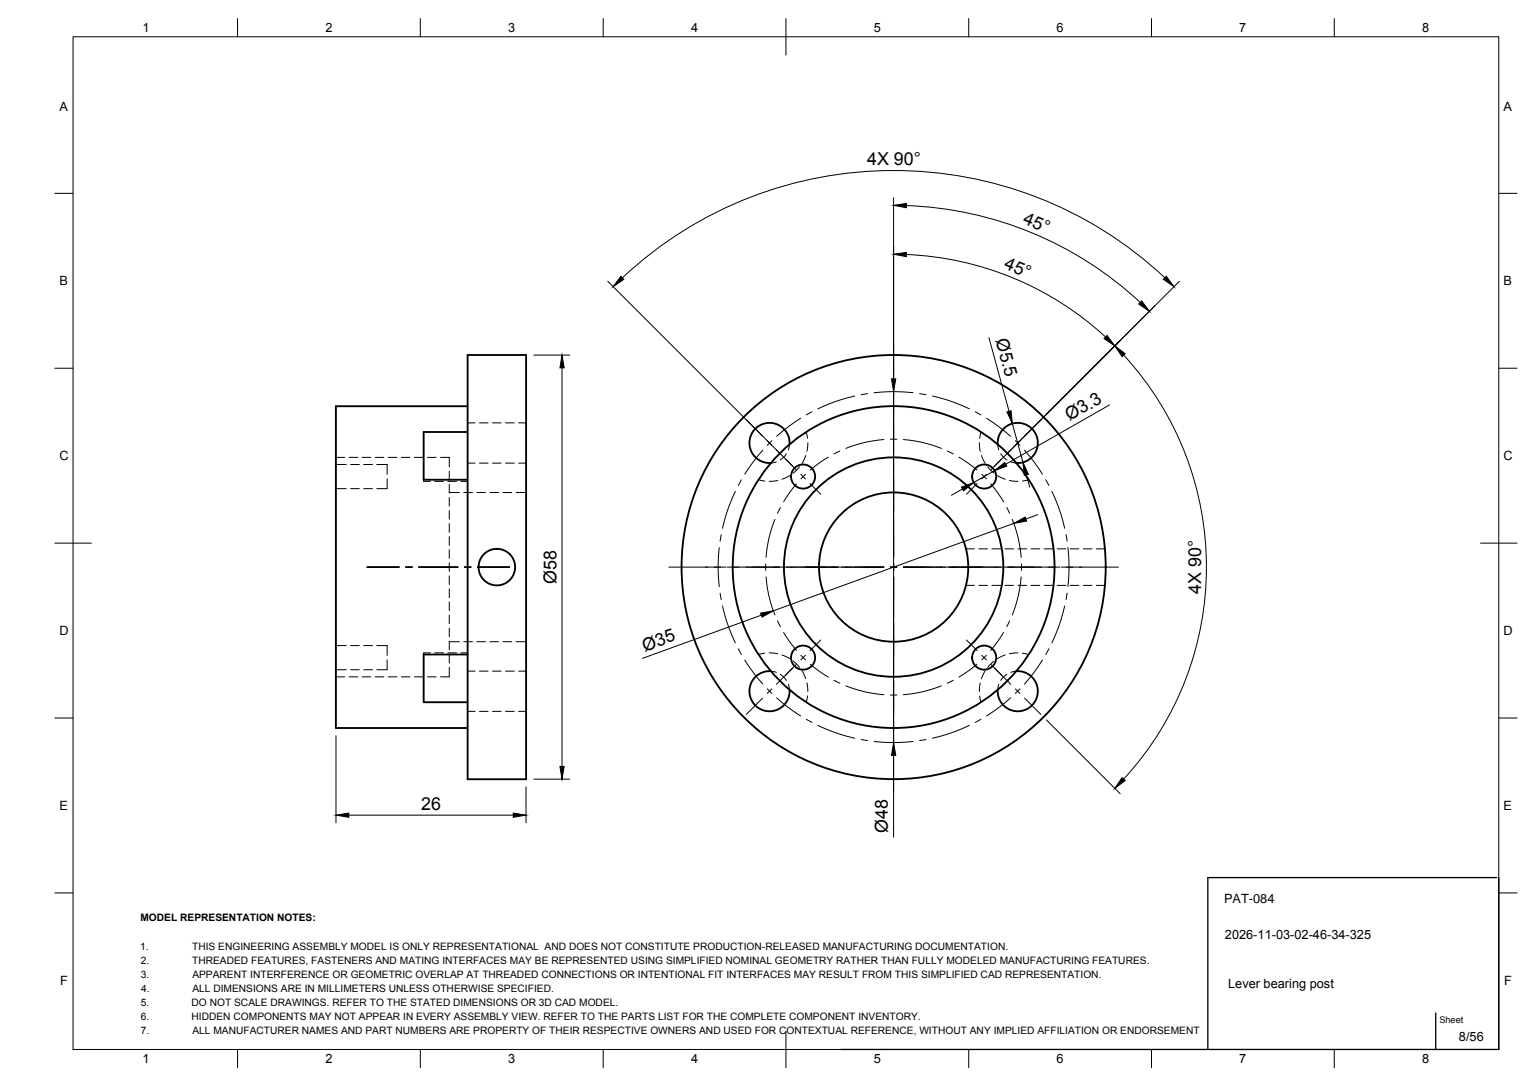
ISO-10303-21;
HEADER;
/* Generated by software containing ST-Developer
 * from STEP Tools, Inc. (www.steptools.com) 
 */

FILE_DESCRIPTION(
/* description */ ('Quick-return (Whitworth) mechanism'),
/* implementation_level */ '2;1');

FILE_NAME(
/* name */ 'Lever bearing post.step',
/* time_stamp */ '2026-10-28T03:25:57-07:00',
/* author */ (''),
/* organization */ (''),
/* preprocessor_version */ 'ST-DEVELOPER v20.2',
/* originating_system */ 'Autodesk Translation Framework v15.17.0.0',
/* authorisation */ '');

FILE_SCHEMA (('AUTOMOTIVE_DESIGN { 1 0 10303 214 3 1 1 }'));
ENDSEC;

DATA;
#10=MECHANICAL_DESIGN_GEOMETRIC_PRESENTATION_REPRESENTATION('',(#493),#14878);
#366=B_SPLINE_CURVE_WITH_KNOTS('',3,(#12105,#12106,#12107,#12108,#12109,
#12110,#12111,#12112,#12113,#12114),.UNSPECIFIED.,.F.,.F.,(4,2,2,2,4),(0.,
0.0945941824764479,0.189188364952896,0.283770357603024,0.378352350253152),
 .UNSPECIFIED.);
#367=B_SPLINE_CURVE_WITH_KNOTS('',3,(#12115,#12116,#12117,#12118,#12119,
#12120,#12121,#12122,#12123,#12124,#12125,#12126,#12127,#12128,#12129,#12130,
#12131,#12132,#12133,#12134,#12135,#12136,#12137,#12138,#12139,#12140),
 .UNSPECIFIED.,.F.,.F.,(4,2,2,2,2,2,2,2,2,2,2,2,4),(0.378352350253152,0.47293434290328,
0.567516335553408,0.662110518029855,0.756704700506303,0.851298882982751,
0.945893065459199,1.04047505810933,1.13505705075946,1.22963904340958,1.32422103605971,
1.41881521853616,1.51340940101261),.UNSPECIFIED.);
#368=B_SPLINE_CURVE_WITH_KNOTS('',3,(#12144,#12145,#12146,#12147,#12148,
#12149,#12150,#12151,#12152,#12153,#12154,#12155,#12156,#12157,#12158,#12159,
#12160,#12161,#12162,#12163,#12164,#12165,#12166,#12167,#12168,#12169),
 .UNSPECIFIED.,.F.,.F.,(4,2,2,2,2,2,2,2,2,2,2,2,4),(0.,0.0942219535700049,
0.18844390714001,0.282665684012033,0.376887460884057,0.471109237756081,
0.565331014628104,0.659552968198109,0.753774921768114,0.847996875338119,
0.942218828908124,1.03644060578015,1.13066238265217),.UNSPECIFIED.);
#369=B_SPLINE_CURVE_WITH_KNOTS('',3,(#12170,#12171,#12172,#12173,#12174,
#12175,#12176,#12177,#12178,#12179),.UNSPECIFIED.,.F.,.F.,(4,2,2,2,4),(1.13066238265217,
1.22488415952419,1.31910593639622,1.41332788996622,1.50754984353623),
 .UNSPECIFIED.);
#405=SHAPE_REPRESENTATION_RELATIONSHIP('SRR','None',#15073,#449);
#449=ADVANCED_BREP_SHAPE_REPRESENTATION('',(#545),#14830);
#493=STYLED_ITEM('',(#15406),#545);
#545=MANIFOLD_SOLID_BREP('Body1',#7847);
#615=FACE_BOUND('',#1585,.T.);
#616=FACE_BOUND('',#1586,.T.);
#617=FACE_BOUND('',#1587,.T.);
#618=FACE_BOUND('',#1588,.T.);
#619=FACE_BOUND('',#1589,.T.);
#620=FACE_BOUND('',#1597,.T.);
#621=FACE_BOUND('',#1599,.T.);
#622=FACE_BOUND('',#1601,.T.);
#623=FACE_BOUND('',#1603,.T.);
#624=FACE_BOUND('',#1604,.T.);
#625=FACE_BOUND('',#1605,.T.);
#626=FACE_BOUND('',#1606,.T.);
#627=FACE_BOUND('',#1607,.T.);
#628=FACE_BOUND('',#1609,.T.);
#629=FACE_BOUND('',#1610,.T.);
#630=FACE_BOUND('',#1611,.T.);
#631=FACE_BOUND('',#1612,.T.);
#632=FACE_BOUND('',#1613,.T.);
#800=PLANE('',#8448);
#801=PLANE('',#8452);
#802=PLANE('',#8456);
#803=PLANE('',#8460);
#804=PLANE('',#8464);
#805=PLANE('',#8469);
#806=PLANE('',#8474);
#807=PLANE('',#8479);
#808=PLANE('',#8481);
#809=PLANE('',#8505);
#810=PLANE('',#8511);
#811=PLANE('',#8512);
#1077=FACE_OUTER_BOUND('',#1567,.T.);
#1078=FACE_OUTER_BOUND('',#1568,.T.);
#1079=FACE_OUTER_BOUND('',#1569,.T.);
#1080=FACE_OUTER_BOUND('',#1570,.T.);
#1081=FACE_OUTER_BOUND('',#1571,.T.);
#1082=FACE_OUTER_BOUND('',#1572,.T.);
#1083=FACE_OUTER_BOUND('',#1573,.T.);
#1084=FACE_OUTER_BOUND('',#1574,.T.);
#1085=FACE_OUTER_BOUND('',#1575,.T.);
#1086=FACE_OUTER_BOUND('',#1576,.T.);
#1087=FACE_OUTER_BOUND('',#1577,.T.);
#1088=FACE_OUTER_BOUND('',#1578,.T.);
#1089=FACE_OUTER_BOUND('',#1579,.T.);
#1090=FACE_OUTER_BOUND('',#1580,.T.);
#1091=FACE_OUTER_BOUND('',#1581,.T.);
#1092=FACE_OUTER_BOUND('',#1582,.T.);
#1093=FACE_OUTER_BOUND('',#1583,.T.);
#1094=FACE_OUTER_BOUND('',#1584,.T.);
#1095=FACE_OUTER_BOUND('',#1590,.T.);
#1096=FACE_OUTER_BOUND('',#1591,.T.);
#1097=FACE_OUTER_BOUND('',#1592,.T.);
#1098=FACE_OUTER_BOUND('',#1593,.T.);
#1099=FACE_OUTER_BOUND('',#1594,.T.);
#1100=FACE_OUTER_BOUND('',#1595,.T.);
#1101=FACE_OUTER_BOUND('',#1596,.T.);
#1102=FACE_OUTER_BOUND('',#1598,.T.);
#1103=FACE_OUTER_BOUND('',#1600,.T.);
#1104=FACE_OUTER_BOUND('',#1602,.T.);
#1105=FACE_OUTER_BOUND('',#1608,.T.);
#1567=EDGE_LOOP('',(#5406,#5407,#5408,#5409,#5410,#5411));
#1568=EDGE_LOOP('',(#5412,#5413,#5414,#5415));
#1569=EDGE_LOOP('',(#5416));
#1570=EDGE_LOOP('',(#5417,#5418,#5419,#5420));
#1571=EDGE_LOOP('',(#5421));
#1572=EDGE_LOOP('',(#5422,#5423,#5424,#5425));
#1573=EDGE_LOOP('',(#5426));
#1574=EDGE_LOOP('',(#5427,#5428,#5429,#5430));
#1575=EDGE_LOOP('',(#5431));
#1576=EDGE_LOOP('',(#5432,#5433,#5434,#5435));
#1577=EDGE_LOOP('',(#5436,#5437));
#1578=EDGE_LOOP('',(#5438,#5439,#5440,#5441));
#1579=EDGE_LOOP('',(#5442,#5443));
#1580=EDGE_LOOP('',(#5444,#5445,#5446,#5447));
#1581=EDGE_LOOP('',(#5448,#5449));
#1582=EDGE_LOOP('',(#5450,#5451,#5452,#5453));
#1583=EDGE_LOOP('',(#5454,#5455));
#1584=EDGE_LOOP('',(#5456));
#1585=EDGE_LOOP('',(#5457,#5458,#5459,#5460,#5461,#5462,#5463,#5464,#5465));
#1586=EDGE_LOOP('',(#5466));
#1587=EDGE_LOOP('',(#5467));
#1588=EDGE_LOOP('',(#5468));
#1589=EDGE_LOOP('',(#5469));
#1590=EDGE_LOOP('',(#5470,#5471,#5472,#5473));
#1591=EDGE_LOOP('',(#5474,#5475,#5476,#5477));
#1592=EDGE_LOOP('',(#5478,#5479,#5480,#5481));
#1593=EDGE_LOOP('',(#5482,#5483,#5484,#5485));
#1594=EDGE_LOOP('',(#5486,#5487,#5488,#5489,#5490,#5491,#5492,#5493,#5494,
#5495,#5496,#5497,#5498,#5499,#5500,#5501,#5502,#5503,#5504,#5505));
#1595=EDGE_LOOP('',(#5506,#5507,#5508,#5509));
#1596=EDGE_LOOP('',(#5510));
#1597=EDGE_LOOP('',(#5511));
#1598=EDGE_LOOP('',(#5512,#5513,#5514,#5515));
#1599=EDGE_LOOP('',(#5516,#5517));
#1600=EDGE_LOOP('',(#5518,#5519,#5520,#5521));
#1601=EDGE_LOOP('',(#5522,#5523));
#1602=EDGE_LOOP('',(#5524));
#1603=EDGE_LOOP('',(#5525));
#1604=EDGE_LOOP('',(#5526));
#1605=EDGE_LOOP('',(#5527));
#1606=EDGE_LOOP('',(#5528));
#1607=EDGE_LOOP('',(#5529));
#1608=EDGE_LOOP('',(#5530));
#1609=EDGE_LOOP('',(#5531));
#1610=EDGE_LOOP('',(#5532));
#1611=EDGE_LOOP('',(#5533));
#1612=EDGE_LOOP('',(#5534));
#1613=EDGE_LOOP('',(#5535));
#2218=LINE('',#12142,#2741);
#2219=LINE('',#12184,#2742);
#2220=LINE('',#12191,#2743);
#2221=LINE('',#12198,#2744);
#2222=LINE('',#12205,#2745);
#2223=LINE('',#12211,#2746);
#2224=LINE('',#12215,#2747);
#2225=LINE('',#12222,#2748);
#2226=LINE('',#12226,#2749);
#2227=LINE('',#12233,#2750);
#2228=LINE('',#12237,#2751);
#2229=LINE('',#12244,#2752);
#2230=LINE('',#12248,#2753);
#2231=LINE('',#12272,#2754);
#2232=LINE('',#12276,#2755);
#2233=LINE('',#12280,#2756);
#2234=LINE('',#12284,#2757);
#2235=LINE('',#12288,#2758);
#2236=LINE('',#12293,#2759);
#2237=LINE('',#12300,#2760);
#2238=LINE('',#12304,#2761);
#2741=VECTOR('',#9567,0.25);
#2742=VECTOR('',#9572,0.165);
#2743=VECTOR('',#9581,0.165);
#2744=VECTOR('',#9590,0.165);
#2745=VECTOR('',#9599,0.165);
#2746=VECTOR('',#9606,1.);
#2747=VECTOR('',#9609,1.);
#2748=VECTOR('',#9618,1.);
#2749=VECTOR('',#9621,1.);
#2750=VECTOR('',#9630,1.);
#2751=VECTOR('',#9633,1.);
#2752=VECTOR('',#9642,1.);
#2753=VECTOR('',#9645,1.);
#2754=VECTOR('',#9678,0.275);
#2755=VECTOR('',#9683,0.275);
#2756=VECTOR('',#9688,0.275);
#2757=VECTOR('',#9693,0.275);
#2758=VECTOR('',#9698,2.2);
#2759=VECTOR('',#9703,1.5);
#2760=VECTOR('',#9712,2.9);
#2761=VECTOR('',#9717,1.02);
#3240=CIRCLE('',#8446,0.165);
#3241=CIRCLE('',#8447,0.165);
#3242=CIRCLE('',#8450,0.165);
#3243=CIRCLE('',#8451,0.165);
#3244=CIRCLE('',#8454,0.165);
#3245=CIRCLE('',#8455,0.165);
#3246=CIRCLE('',#8458,0.165);
#3247=CIRCLE('',#8459,0.165);
#3248=CIRCLE('',#8462,0.525);
#3249=CIRCLE('',#8463,0.525);
#3250=CIRCLE('',#8465,2.2);
#3251=CIRCLE('',#8467,0.525);
#3252=CIRCLE('',#8468,0.525);
#3253=CIRCLE('',#8470,2.2);
#3254=CIRCLE('',#8472,0.525);
#3255=CIRCLE('',#8473,0.525);
#3256=CIRCLE('',#8475,2.2);
#3257=CIRCLE('',#8477,0.525);
#3258=CIRCLE('',#8478,0.525);
#3259=CIRCLE('',#8480,2.2);
#3260=CIRCLE('',#8482,2.9);
#3261=CIRCLE('',#8483,2.2);
#3262=CIRCLE('',#8484,2.2);
#3263=CIRCLE('',#8485,2.2);
#3264=CIRCLE('',#8486,2.2);
#3265=CIRCLE('',#8487,2.2);
#3266=CIRCLE('',#8488,0.275);
#3267=CIRCLE('',#8489,0.275);
#3268=CIRCLE('',#8490,0.275);
#3269=CIRCLE('',#8491,0.275);
#3270=CIRCLE('',#8493,0.275);
#3271=CIRCLE('',#8495,0.275);
#3272=CIRCLE('',#8497,0.275);
#3273=CIRCLE('',#8499,0.275);
#3274=CIRCLE('',#8501,2.2);
#3275=CIRCLE('',#8503,1.5);
#3276=CIRCLE('',#8504,1.5);
#3277=CIRCLE('',#8506,1.02);
#3278=CIRCLE('',#8508,2.9);
#3279=CIRCLE('',#8510,1.02);
#3679=VERTEX_POINT('',#12103);
#3680=VERTEX_POINT('',#12104);
#3681=VERTEX_POINT('',#12141);
#3682=VERTEX_POINT('',#12143);
#3683=VERTEX_POINT('',#12181);
#3684=VERTEX_POINT('',#12183);
#3685=VERTEX_POINT('',#12188);
#3686=VERTEX_POINT('',#12190);
#3687=VERTEX_POINT('',#12195);
#3688=VERTEX_POINT('',#12197);
#3689=VERTEX_POINT('',#12202);
#3690=VERTEX_POINT('',#12204);
#3691=VERTEX_POINT('',#12209);
#3692=VERTEX_POINT('',#12210);
#3693=VERTEX_POINT('',#12212);
#3694=VERTEX_POINT('',#12214);
#3695=VERTEX_POINT('',#12220);
#3696=VERTEX_POINT('',#12221);
#3697=VERTEX_POINT('',#12223);
#3698=VERTEX_POINT('',#12225);
#3699=VERTEX_POINT('',#12231);
#3700=VERTEX_POINT('',#12232);
#3701=VERTEX_POINT('',#12234);
#3702=VERTEX_POINT('',#12236);
#3703=VERTEX_POINT('',#12242);
#3704=VERTEX_POINT('',#12243);
#3705=VERTEX_POINT('',#12245);
#3706=VERTEX_POINT('',#12247);
#3707=VERTEX_POINT('',#12253);
#3708=VERTEX_POINT('',#12255);
#3709=VERTEX_POINT('',#12261);
#3710=VERTEX_POINT('',#12263);
#3711=VERTEX_POINT('',#12265);
#3712=VERTEX_POINT('',#12267);
#3713=VERTEX_POINT('',#12270);
#3714=VERTEX_POINT('',#12274);
#3715=VERTEX_POINT('',#12278);
#3716=VERTEX_POINT('',#12282);
#3717=VERTEX_POINT('',#12286);
#3718=VERTEX_POINT('',#12290);
#3719=VERTEX_POINT('',#12292);
#3720=VERTEX_POINT('',#12296);
#3721=VERTEX_POINT('',#12299);
#3722=VERTEX_POINT('',#12303);
#4360=EDGE_CURVE('',#3679,#3680,#366,.T.);
#4361=EDGE_CURVE('',#3680,#3679,#367,.T.);
#4362=EDGE_CURVE('',#3680,#3681,#2218,.T.);
#4363=EDGE_CURVE('',#3682,#3681,#368,.T.);
#4364=EDGE_CURVE('',#3681,#3682,#369,.T.);
#4365=EDGE_CURVE('',#3683,#3683,#3240,.T.);
#4366=EDGE_CURVE('',#3683,#3684,#2219,.T.);
#4367=EDGE_CURVE('',#3684,#3684,#3241,.T.);
#4368=EDGE_CURVE('',#3685,#3685,#3242,.T.);
#4369=EDGE_CURVE('',#3685,#3686,#2220,.T.);
#4370=EDGE_CURVE('',#3686,#3686,#3243,.T.);
#4371=EDGE_CURVE('',#3687,#3687,#3244,.T.);
#4372=EDGE_CURVE('',#3687,#3688,#2221,.T.);
#4373=EDGE_CURVE('',#3688,#3688,#3245,.T.);
#4374=EDGE_CURVE('',#3689,#3689,#3246,.T.);
#4375=EDGE_CURVE('',#3689,#3690,#2222,.T.);
#4376=EDGE_CURVE('',#3690,#3690,#3247,.T.);
#4377=EDGE_CURVE('',#3691,#3692,#2223,.T.);
#4378=EDGE_CURVE('',#3691,#3693,#3248,.T.);
#4379=EDGE_CURVE('',#3694,#3693,#2224,.T.);
#4380=EDGE_CURVE('',#3692,#3694,#3249,.T.);
#4381=EDGE_CURVE('',#3693,#3691,#3250,.T.);
#4382=EDGE_CURVE('',#3695,#3696,#2225,.T.);
#4383=EDGE_CURVE('',#3695,#3697,#3251,.T.);
#4384=EDGE_CURVE('',#3698,#3697,#2226,.T.);
#4385=EDGE_CURVE('',#3696,#3698,#3252,.T.);
#4386=EDGE_CURVE('',#3697,#3695,#3253,.T.);
#4387=EDGE_CURVE('',#3699,#3700,#2227,.T.);
#4388=EDGE_CURVE('',#3699,#3701,#3254,.T.);
#4389=EDGE_CURVE('',#3702,#3701,#2228,.T.);
#4390=EDGE_CURVE('',#3700,#3702,#3255,.T.);
#4391=EDGE_CURVE('',#3701,#3699,#3256,.T.);
#4392=EDGE_CURVE('',#3703,#3704,#2229,.T.);
#4393=EDGE_CURVE('',#3703,#3705,#3257,.T.);
#4394=EDGE_CURVE('',#3706,#3705,#2230,.T.);
#4395=EDGE_CURVE('',#3704,#3706,#3258,.T.);
#4396=EDGE_CURVE('',#3705,#3703,#3259,.T.);
#4397=EDGE_CURVE('',#3707,#3707,#3260,.T.);
#4398=EDGE_CURVE('',#3696,#3708,#3261,.T.);
#4399=EDGE_CURVE('',#3700,#3698,#3262,.T.);
#4400=EDGE_CURVE('',#3704,#3702,#3263,.T.);
#4401=EDGE_CURVE('',#3692,#3706,#3264,.T.);
#4402=EDGE_CURVE('',#3708,#3694,#3265,.T.);
#4403=EDGE_CURVE('',#3709,#3709,#3266,.T.);
#4404=EDGE_CURVE('',#3710,#3710,#3267,.T.);
#4405=EDGE_CURVE('',#3711,#3711,#3268,.T.);
#4406=EDGE_CURVE('',#3712,#3712,#3269,.T.);
#4407=EDGE_CURVE('',#3713,#3713,#3270,.T.);
#4408=EDGE_CURVE('',#3713,#3709,#2231,.T.);
#4409=EDGE_CURVE('',#3714,#3714,#3271,.T.);
#4410=EDGE_CURVE('',#3714,#3710,#2232,.T.);
#4411=EDGE_CURVE('',#3715,#3715,#3272,.T.);
#4412=EDGE_CURVE('',#3715,#3711,#2233,.T.);
#4413=EDGE_CURVE('',#3716,#3716,#3273,.T.);
#4414=EDGE_CURVE('',#3716,#3712,#2234,.T.);
#4415=EDGE_CURVE('',#3717,#3717,#3274,.T.);
#4416=EDGE_CURVE('',#3717,#3708,#2235,.T.);
#4417=EDGE_CURVE('',#3718,#3718,#3275,.T.);
#4418=EDGE_CURVE('',#3718,#3719,#2236,.T.);
#4419=EDGE_CURVE('',#3719,#3719,#3276,.T.);
#4420=EDGE_CURVE('',#3720,#3720,#3277,.T.);
#4421=EDGE_CURVE('',#3707,#3721,#2237,.T.);
#4422=EDGE_CURVE('',#3721,#3721,#3278,.T.);
#4423=EDGE_CURVE('',#3720,#3722,#2238,.T.);
#4424=EDGE_CURVE('',#3722,#3722,#3279,.T.);
#5406=ORIENTED_EDGE('',*,*,#4360,.F.);
#5407=ORIENTED_EDGE('',*,*,#4361,.F.);
#5408=ORIENTED_EDGE('',*,*,#4362,.T.);
#5409=ORIENTED_EDGE('',*,*,#4363,.F.);
#5410=ORIENTED_EDGE('',*,*,#4364,.F.);
#5411=ORIENTED_EDGE('',*,*,#4362,.F.);
#5412=ORIENTED_EDGE('',*,*,#4365,.F.);
#5413=ORIENTED_EDGE('',*,*,#4366,.T.);
#5414=ORIENTED_EDGE('',*,*,#4367,.F.);
#5415=ORIENTED_EDGE('',*,*,#4366,.F.);
#5416=ORIENTED_EDGE('',*,*,#4365,.T.);
#5417=ORIENTED_EDGE('',*,*,#4368,.F.);
#5418=ORIENTED_EDGE('',*,*,#4369,.T.);
#5419=ORIENTED_EDGE('',*,*,#4370,.F.);
#5420=ORIENTED_EDGE('',*,*,#4369,.F.);
#5421=ORIENTED_EDGE('',*,*,#4368,.T.);
#5422=ORIENTED_EDGE('',*,*,#4371,.F.);
#5423=ORIENTED_EDGE('',*,*,#4372,.T.);
#5424=ORIENTED_EDGE('',*,*,#4373,.F.);
#5425=ORIENTED_EDGE('',*,*,#4372,.F.);
#5426=ORIENTED_EDGE('',*,*,#4371,.T.);
#5427=ORIENTED_EDGE('',*,*,#4374,.F.);
#5428=ORIENTED_EDGE('',*,*,#4375,.T.);
#5429=ORIENTED_EDGE('',*,*,#4376,.F.);
#5430=ORIENTED_EDGE('',*,*,#4375,.F.);
#5431=ORIENTED_EDGE('',*,*,#4374,.T.);
#5432=ORIENTED_EDGE('',*,*,#4377,.F.);
#5433=ORIENTED_EDGE('',*,*,#4378,.T.);
#5434=ORIENTED_EDGE('',*,*,#4379,.F.);
#5435=ORIENTED_EDGE('',*,*,#4380,.F.);
#5436=ORIENTED_EDGE('',*,*,#4381,.F.);
#5437=ORIENTED_EDGE('',*,*,#4378,.F.);
#5438=ORIENTED_EDGE('',*,*,#4382,.F.);
#5439=ORIENTED_EDGE('',*,*,#4383,.T.);
#5440=ORIENTED_EDGE('',*,*,#4384,.F.);
#5441=ORIENTED_EDGE('',*,*,#4385,.F.);
#5442=ORIENTED_EDGE('',*,*,#4386,.F.);
#5443=ORIENTED_EDGE('',*,*,#4383,.F.);
#5444=ORIENTED_EDGE('',*,*,#4387,.F.);
#5445=ORIENTED_EDGE('',*,*,#4388,.T.);
#5446=ORIENTED_EDGE('',*,*,#4389,.F.);
#5447=ORIENTED_EDGE('',*,*,#4390,.F.);
#5448=ORIENTED_EDGE('',*,*,#4391,.F.);
#5449=ORIENTED_EDGE('',*,*,#4388,.F.);
#5450=ORIENTED_EDGE('',*,*,#4392,.F.);
#5451=ORIENTED_EDGE('',*,*,#4393,.T.);
#5452=ORIENTED_EDGE('',*,*,#4394,.F.);
#5453=ORIENTED_EDGE('',*,*,#4395,.F.);
#5454=ORIENTED_EDGE('',*,*,#4396,.F.);
#5455=ORIENTED_EDGE('',*,*,#4393,.F.);
#5456=ORIENTED_EDGE('',*,*,#4397,.T.);
#5457=ORIENTED_EDGE('',*,*,#4398,.F.);
#5458=ORIENTED_EDGE('',*,*,#4385,.T.);
#5459=ORIENTED_EDGE('',*,*,#4399,.F.);
#5460=ORIENTED_EDGE('',*,*,#4390,.T.);
#5461=ORIENTED_EDGE('',*,*,#4400,.F.);
#5462=ORIENTED_EDGE('',*,*,#4395,.T.);
#5463=ORIENTED_EDGE('',*,*,#4401,.F.);
#5464=ORIENTED_EDGE('',*,*,#4380,.T.);
#5465=ORIENTED_EDGE('',*,*,#4402,.F.);
#5466=ORIENTED_EDGE('',*,*,#4403,.T.);
#5467=ORIENTED_EDGE('',*,*,#4404,.T.);
#5468=ORIENTED_EDGE('',*,*,#4405,.T.);
#5469=ORIENTED_EDGE('',*,*,#4406,.T.);
#5470=ORIENTED_EDGE('',*,*,#4407,.F.);
#5471=ORIENTED_EDGE('',*,*,#4408,.T.);
#5472=ORIENTED_EDGE('',*,*,#4403,.F.);
#5473=ORIENTED_EDGE('',*,*,#4408,.F.);
#5474=ORIENTED_EDGE('',*,*,#4409,.F.);
#5475=ORIENTED_EDGE('',*,*,#4410,.T.);
#5476=ORIENTED_EDGE('',*,*,#4404,.F.);
#5477=ORIENTED_EDGE('',*,*,#4410,.F.);
#5478=ORIENTED_EDGE('',*,*,#4411,.F.);
#5479=ORIENTED_EDGE('',*,*,#4412,.T.);
#5480=ORIENTED_EDGE('',*,*,#4405,.F.);
#5481=ORIENTED_EDGE('',*,*,#4412,.F.);
#5482=ORIENTED_EDGE('',*,*,#4413,.F.);
#5483=ORIENTED_EDGE('',*,*,#4414,.T.);
#5484=ORIENTED_EDGE('',*,*,#4406,.F.);
#5485=ORIENTED_EDGE('',*,*,#4414,.F.);
#5486=ORIENTED_EDGE('',*,*,#4415,.F.);
#5487=ORIENTED_EDGE('',*,*,#4416,.T.);
#5488=ORIENTED_EDGE('',*,*,#4402,.T.);
#5489=ORIENTED_EDGE('',*,*,#4379,.T.);
#5490=ORIENTED_EDGE('',*,*,#4381,.T.);
#5491=ORIENTED_EDGE('',*,*,#4377,.T.);
#5492=ORIENTED_EDGE('',*,*,#4401,.T.);
#5493=ORIENTED_EDGE('',*,*,#4394,.T.);
#5494=ORIENTED_EDGE('',*,*,#4396,.T.);
#5495=ORIENTED_EDGE('',*,*,#4392,.T.);
#5496=ORIENTED_EDGE('',*,*,#4400,.T.);
#5497=ORIENTED_EDGE('',*,*,#4389,.T.);
#5498=ORIENTED_EDGE('',*,*,#4391,.T.);
#5499=ORIENTED_EDGE('',*,*,#4387,.T.);
#5500=ORIENTED_EDGE('',*,*,#4399,.T.);
#5501=ORIENTED_EDGE('',*,*,#4384,.T.);
#5502=ORIENTED_EDGE('',*,*,#4386,.T.);
#5503=ORIENTED_EDGE('',*,*,#4382,.T.);
#5504=ORIENTED_EDGE('',*,*,#4398,.T.);
#5505=ORIENTED_EDGE('',*,*,#4416,.F.);
#5506=ORIENTED_EDGE('',*,*,#4417,.F.);
#5507=ORIENTED_EDGE('',*,*,#4418,.T.);
#5508=ORIENTED_EDGE('',*,*,#4419,.F.);
#5509=ORIENTED_EDGE('',*,*,#4418,.F.);
#5510=ORIENTED_EDGE('',*,*,#4417,.T.);
#5511=ORIENTED_EDGE('',*,*,#4420,.F.);
#5512=ORIENTED_EDGE('',*,*,#4397,.F.);
#5513=ORIENTED_EDGE('',*,*,#4421,.T.);
#5514=ORIENTED_EDGE('',*,*,#4422,.T.);
#5515=ORIENTED_EDGE('',*,*,#4421,.F.);
#5516=ORIENTED_EDGE('',*,*,#4363,.T.);
#5517=ORIENTED_EDGE('',*,*,#4364,.T.);
#5518=ORIENTED_EDGE('',*,*,#4420,.T.);
#5519=ORIENTED_EDGE('',*,*,#4423,.T.);
#5520=ORIENTED_EDGE('',*,*,#4424,.T.);
#5521=ORIENTED_EDGE('',*,*,#4423,.F.);
#5522=ORIENTED_EDGE('',*,*,#4360,.T.);
#5523=ORIENTED_EDGE('',*,*,#4361,.T.);
#5524=ORIENTED_EDGE('',*,*,#4415,.T.);
#5525=ORIENTED_EDGE('',*,*,#4419,.T.);
#5526=ORIENTED_EDGE('',*,*,#4376,.T.);
#5527=ORIENTED_EDGE('',*,*,#4373,.T.);
#5528=ORIENTED_EDGE('',*,*,#4370,.T.);
#5529=ORIENTED_EDGE('',*,*,#4367,.T.);
#5530=ORIENTED_EDGE('',*,*,#4422,.F.);
#5531=ORIENTED_EDGE('',*,*,#4424,.F.);
#5532=ORIENTED_EDGE('',*,*,#4413,.T.);
#5533=ORIENTED_EDGE('',*,*,#4411,.T.);
#5534=ORIENTED_EDGE('',*,*,#4409,.T.);
#5535=ORIENTED_EDGE('',*,*,#4407,.T.);
#7222=CYLINDRICAL_SURFACE('',#8444,0.25);
#7223=CYLINDRICAL_SURFACE('',#8445,0.165);
#7224=CYLINDRICAL_SURFACE('',#8449,0.165);
#7225=CYLINDRICAL_SURFACE('',#8453,0.165);
#7226=CYLINDRICAL_SURFACE('',#8457,0.165);
#7227=CYLINDRICAL_SURFACE('',#8461,0.525);
#7228=CYLINDRICAL_SURFACE('',#8466,0.525);
#7229=CYLINDRICAL_SURFACE('',#8471,0.525);
#7230=CYLINDRICAL_SURFACE('',#8476,0.525);
#7231=CYLINDRICAL_SURFACE('',#8492,0.275);
#7232=CYLINDRICAL_SURFACE('',#8494,0.275);
#7233=CYLINDRICAL_SURFACE('',#8496,0.275);
#7234=CYLINDRICAL_SURFACE('',#8498,0.275);
#7235=CYLINDRICAL_SURFACE('',#8500,2.2);
#7236=CYLINDRICAL_SURFACE('',#8502,1.5);
#7237=CYLINDRICAL_SURFACE('',#8507,2.9);
#7238=CYLINDRICAL_SURFACE('',#8509,1.02);
#7408=ADVANCED_FACE('',(#1077),#7222,.F.);
#7409=ADVANCED_FACE('',(#1078),#7223,.F.);
#7410=ADVANCED_FACE('',(#1079),#800,.T.);
#7411=ADVANCED_FACE('',(#1080),#7224,.F.);
#7412=ADVANCED_FACE('',(#1081),#801,.T.);
#7413=ADVANCED_FACE('',(#1082),#7225,.F.);
#7414=ADVANCED_FACE('',(#1083),#802,.T.);
#7415=ADVANCED_FACE('',(#1084),#7226,.F.);
#7416=ADVANCED_FACE('',(#1085),#803,.T.);
#7417=ADVANCED_FACE('',(#1086),#7227,.F.);
#7418=ADVANCED_FACE('',(#1087),#804,.F.);
#7419=ADVANCED_FACE('',(#1088),#7228,.F.);
#7420=ADVANCED_FACE('',(#1089),#805,.F.);
#7421=ADVANCED_FACE('',(#1090),#7229,.F.);
#7422=ADVANCED_FACE('',(#1091),#806,.F.);
#7423=ADVANCED_FACE('',(#1092),#7230,.F.);
#7424=ADVANCED_FACE('',(#1093),#807,.F.);
#7425=ADVANCED_FACE('',(#1094,#615,#616,#617,#618,#619),#808,.T.);
#7426=ADVANCED_FACE('',(#1095),#7231,.F.);
#7427=ADVANCED_FACE('',(#1096),#7232,.F.);
#7428=ADVANCED_FACE('',(#1097),#7233,.F.);
#7429=ADVANCED_FACE('',(#1098),#7234,.F.);
#7430=ADVANCED_FACE('',(#1099),#7235,.T.);
#7431=ADVANCED_FACE('',(#1100),#7236,.F.);
#7432=ADVANCED_FACE('',(#1101,#620),#809,.T.);
#7433=ADVANCED_FACE('',(#1102,#621),#7237,.T.);
#7434=ADVANCED_FACE('',(#1103,#622),#7238,.F.);
#7435=ADVANCED_FACE('',(#1104,#623,#624,#625,#626,#627),#810,.T.);
#7436=ADVANCED_FACE('',(#1105,#628,#629,#630,#631,#632),#811,.F.);
#7847=CLOSED_SHELL('',(#7408,#7409,#7410,#7411,#7412,#7413,#7414,#7415,
#7416,#7417,#7418,#7419,#7420,#7421,#7422,#7423,#7424,#7425,#7426,#7427,
#7428,#7429,#7430,#7431,#7432,#7433,#7434,#7435,#7436));
#8443=AXIS2_PLACEMENT_3D('',#12101,#9563,#9564);
#8444=AXIS2_PLACEMENT_3D('',#12102,#9565,#9566);
#8445=AXIS2_PLACEMENT_3D('',#12180,#9568,#9569);
#8446=AXIS2_PLACEMENT_3D('',#12182,#9570,#9571);
#8447=AXIS2_PLACEMENT_3D('',#12185,#9573,#9574);
#8448=AXIS2_PLACEMENT_3D('',#12186,#9575,#9576);
#8449=AXIS2_PLACEMENT_3D('',#12187,#9577,#9578);
#8450=AXIS2_PLACEMENT_3D('',#12189,#9579,#9580);
#8451=AXIS2_PLACEMENT_3D('',#12192,#9582,#9583);
#8452=AXIS2_PLACEMENT_3D('',#12193,#9584,#9585);
#8453=AXIS2_PLACEMENT_3D('',#12194,#9586,#9587);
#8454=AXIS2_PLACEMENT_3D('',#12196,#9588,#9589);
#8455=AXIS2_PLACEMENT_3D('',#12199,#9591,#9592);
#8456=AXIS2_PLACEMENT_3D('',#12200,#9593,#9594);
#8457=AXIS2_PLACEMENT_3D('',#12201,#9595,#9596);
#8458=AXIS2_PLACEMENT_3D('',#12203,#9597,#9598);
#8459=AXIS2_PLACEMENT_3D('',#12206,#9600,#9601);
#8460=AXIS2_PLACEMENT_3D('',#12207,#9602,#9603);
#8461=AXIS2_PLACEMENT_3D('',#12208,#9604,#9605);
#8462=AXIS2_PLACEMENT_3D('',#12213,#9607,#9608);
#8463=AXIS2_PLACEMENT_3D('',#12216,#9610,#9611);
#8464=AXIS2_PLACEMENT_3D('',#12217,#9612,#9613);
#8465=AXIS2_PLACEMENT_3D('',#12218,#9614,#9615);
#8466=AXIS2_PLACEMENT_3D('',#12219,#9616,#9617);
#8467=AXIS2_PLACEMENT_3D('',#12224,#9619,#9620);
#8468=AXIS2_PLACEMENT_3D('',#12227,#9622,#9623);
#8469=AXIS2_PLACEMENT_3D('',#12228,#9624,#9625);
#8470=AXIS2_PLACEMENT_3D('',#12229,#9626,#9627);
#8471=AXIS2_PLACEMENT_3D('',#12230,#9628,#9629);
#8472=AXIS2_PLACEMENT_3D('',#12235,#9631,#9632);
#8473=AXIS2_PLACEMENT_3D('',#12238,#9634,#9635);
#8474=AXIS2_PLACEMENT_3D('',#12239,#9636,#9637);
#8475=AXIS2_PLACEMENT_3D('',#12240,#9638,#9639);
#8476=AXIS2_PLACEMENT_3D('',#12241,#9640,#9641);
#8477=AXIS2_PLACEMENT_3D('',#12246,#9643,#9644);
#8478=AXIS2_PLACEMENT_3D('',#12249,#9646,#9647);
#8479=AXIS2_PLACEMENT_3D('',#12250,#9648,#9649);
#8480=AXIS2_PLACEMENT_3D('',#12251,#9650,#9651);
#8481=AXIS2_PLACEMENT_3D('',#12252,#9652,#9653);
#8482=AXIS2_PLACEMENT_3D('',#12254,#9654,#9655);
#8483=AXIS2_PLACEMENT_3D('',#12256,#9656,#9657);
#8484=AXIS2_PLACEMENT_3D('',#12257,#9658,#9659);
#8485=AXIS2_PLACEMENT_3D('',#12258,#9660,#9661);
#8486=AXIS2_PLACEMENT_3D('',#12259,#9662,#9663);
#8487=AXIS2_PLACEMENT_3D('',#12260,#9664,#9665);
#8488=AXIS2_PLACEMENT_3D('',#12262,#9666,#9667);
#8489=AXIS2_PLACEMENT_3D('',#12264,#9668,#9669);
#8490=AXIS2_PLACEMENT_3D('',#12266,#9670,#9671);
#8491=AXIS2_PLACEMENT_3D('',#12268,#9672,#9673);
#8492=AXIS2_PLACEMENT_3D('',#12269,#9674,#9675);
#8493=AXIS2_PLACEMENT_3D('',#12271,#9676,#9677);
#8494=AXIS2_PLACEMENT_3D('',#12273,#9679,#9680);
#8495=AXIS2_PLACEMENT_3D('',#12275,#9681,#9682);
#8496=AXIS2_PLACEMENT_3D('',#12277,#9684,#9685);
#8497=AXIS2_PLACEMENT_3D('',#12279,#9686,#9687);
#8498=AXIS2_PLACEMENT_3D('',#12281,#9689,#9690);
#8499=AXIS2_PLACEMENT_3D('',#12283,#9691,#9692);
#8500=AXIS2_PLACEMENT_3D('',#12285,#9694,#9695);
#8501=AXIS2_PLACEMENT_3D('',#12287,#9696,#9697);
#8502=AXIS2_PLACEMENT_3D('',#12289,#9699,#9700);
#8503=AXIS2_PLACEMENT_3D('',#12291,#9701,#9702);
#8504=AXIS2_PLACEMENT_3D('',#12294,#9704,#9705);
#8505=AXIS2_PLACEMENT_3D('',#12295,#9706,#9707);
#8506=AXIS2_PLACEMENT_3D('',#12297,#9708,#9709);
#8507=AXIS2_PLACEMENT_3D('',#12298,#9710,#9711);
#8508=AXIS2_PLACEMENT_3D('',#12301,#9713,#9714);
#8509=AXIS2_PLACEMENT_3D('',#12302,#9715,#9716);
#8510=AXIS2_PLACEMENT_3D('',#12305,#9718,#9719);
#8511=AXIS2_PLACEMENT_3D('',#12306,#9720,#9721);
#8512=AXIS2_PLACEMENT_3D('',#12307,#9722,#9723);
#9563=DIRECTION('axis',(0.,0.,1.));
#9564=DIRECTION('refdir',(1.,0.,0.));
#9565=DIRECTION('center_axis',(1.,0.,0.));
#9566=DIRECTION('ref_axis',(0.,0.,-1.));
#9567=DIRECTION('',(1.,0.,0.));
#9568=DIRECTION('center_axis',(0.,0.,1.));
#9569=DIRECTION('ref_axis',(1.,0.,0.));
#9570=DIRECTION('center_axis',(0.,0.,1.));
#9571=DIRECTION('ref_axis',(1.,0.,0.));
#9572=DIRECTION('',(0.,0.,1.));
#9573=DIRECTION('center_axis',(0.,0.,-1.));
#9574=DIRECTION('ref_axis',(1.,0.,0.));
#9575=DIRECTION('center_axis',(0.,0.,1.));
#9576=DIRECTION('ref_axis',(1.,0.,0.));
#9577=DIRECTION('center_axis',(0.,0.,1.));
#9578=DIRECTION('ref_axis',(1.,0.,0.));
#9579=DIRECTION('center_axis',(0.,0.,1.));
#9580=DIRECTION('ref_axis',(1.,0.,0.));
#9581=DIRECTION('',(0.,0.,1.));
#9582=DIRECTION('center_axis',(0.,0.,-1.));
#9583=DIRECTION('ref_axis',(1.,0.,0.));
#9584=DIRECTION('center_axis',(0.,0.,1.));
#9585=DIRECTION('ref_axis',(1.,0.,0.));
#9586=DIRECTION('center_axis',(0.,0.,1.));
#9587=DIRECTION('ref_axis',(1.,0.,0.));
#9588=DIRECTION('center_axis',(0.,0.,1.));
#9589=DIRECTION('ref_axis',(1.,0.,0.));
#9590=DIRECTION('',(0.,0.,1.));
#9591=DIRECTION('center_axis',(0.,0.,-1.));
#9592=DIRECTION('ref_axis',(1.,0.,0.));
#9593=DIRECTION('center_axis',(0.,0.,1.));
#9594=DIRECTION('ref_axis',(1.,0.,0.));
#9595=DIRECTION('center_axis',(0.,0.,1.));
#9596=DIRECTION('ref_axis',(1.,0.,0.));
#9597=DIRECTION('center_axis',(0.,0.,1.));
#9598=DIRECTION('ref_axis',(1.,0.,0.));
#9599=DIRECTION('',(0.,0.,1.));
#9600=DIRECTION('center_axis',(0.,0.,-1.));
#9601=DIRECTION('ref_axis',(1.,0.,0.));
#9602=DIRECTION('center_axis',(0.,0.,1.));
#9603=DIRECTION('ref_axis',(1.,0.,0.));
#9604=DIRECTION('center_axis',(0.,0.,1.));
#9605=DIRECTION('ref_axis',(1.,0.,0.));
#9606=DIRECTION('',(0.,0.,-1.));
#9607=DIRECTION('center_axis',(0.,0.,1.));
#9608=DIRECTION('ref_axis',(1.,0.,0.));
#9609=DIRECTION('',(0.,0.,1.));
#9610=DIRECTION('center_axis',(0.,0.,1.));
#9611=DIRECTION('ref_axis',(1.,0.,0.));
#9612=DIRECTION('center_axis',(0.,0.,1.));
#9613=DIRECTION('ref_axis',(1.,0.,0.));
#9614=DIRECTION('center_axis',(0.,0.,1.));
#9615=DIRECTION('ref_axis',(1.,0.,0.));
#9616=DIRECTION('center_axis',(0.,0.,1.));
#9617=DIRECTION('ref_axis',(1.,0.,0.));
#9618=DIRECTION('',(0.,0.,-1.));
#9619=DIRECTION('center_axis',(0.,0.,1.));
#9620=DIRECTION('ref_axis',(1.,0.,0.));
#9621=DIRECTION('',(0.,0.,1.));
#9622=DIRECTION('center_axis',(0.,0.,1.));
#9623=DIRECTION('ref_axis',(1.,0.,0.));
#9624=DIRECTION('center_axis',(0.,0.,1.));
#9625=DIRECTION('ref_axis',(1.,0.,0.));
#9626=DIRECTION('center_axis',(0.,0.,1.));
#9627=DIRECTION('ref_axis',(1.,0.,0.));
#9628=DIRECTION('center_axis',(0.,0.,1.));
#9629=DIRECTION('ref_axis',(-0.707106781186548,-0.707106781186547,0.));
#9630=DIRECTION('',(0.,0.,-1.));
#9631=DIRECTION('center_axis',(0.,0.,1.));
#9632=DIRECTION('ref_axis',(1.,0.,0.));
#9633=DIRECTION('',(0.,0.,1.));
#9634=DIRECTION('center_axis',(0.,0.,1.));
#9635=DIRECTION('ref_axis',(1.,0.,0.));
#9636=DIRECTION('center_axis',(0.,0.,1.));
#9637=DIRECTION('ref_axis',(1.,0.,0.));
#9638=DIRECTION('center_axis',(0.,0.,1.));
#9639=DIRECTION('ref_axis',(1.,0.,0.));
#9640=DIRECTION('center_axis',(0.,0.,1.));
#9641=DIRECTION('ref_axis',(-0.707106781186547,0.707106781186548,0.));
#9642=DIRECTION('',(0.,0.,-1.));
#9643=DIRECTION('center_axis',(0.,0.,1.));
#9644=DIRECTION('ref_axis',(1.,0.,0.));
#9645=DIRECTION('',(0.,0.,1.));
#9646=DIRECTION('center_axis',(0.,0.,1.));
#9647=DIRECTION('ref_axis',(1.,0.,0.));
#9648=DIRECTION('center_axis',(0.,0.,1.));
#9649=DIRECTION('ref_axis',(1.,0.,0.));
#9650=DIRECTION('center_axis',(0.,0.,1.));
#9651=DIRECTION('ref_axis',(1.,0.,0.));
#9652=DIRECTION('center_axis',(0.,0.,1.));
#9653=DIRECTION('ref_axis',(1.,0.,0.));
#9654=DIRECTION('center_axis',(0.,0.,1.));
#9655=DIRECTION('ref_axis',(1.,0.,0.));
#9656=DIRECTION('center_axis',(0.,0.,1.));
#9657=DIRECTION('ref_axis',(1.,0.,0.));
#9658=DIRECTION('center_axis',(0.,0.,1.));
#9659=DIRECTION('ref_axis',(1.,0.,0.));
#9660=DIRECTION('center_axis',(0.,0.,1.));
#9661=DIRECTION('ref_axis',(1.,0.,0.));
#9662=DIRECTION('center_axis',(0.,0.,1.));
#9663=DIRECTION('ref_axis',(1.,0.,0.));
#9664=DIRECTION('center_axis',(0.,0.,1.));
#9665=DIRECTION('ref_axis',(1.,0.,0.));
#9666=DIRECTION('center_axis',(0.,0.,-1.));
#9667=DIRECTION('ref_axis',(1.,0.,0.));
#9668=DIRECTION('center_axis',(0.,0.,-1.));
#9669=DIRECTION('ref_axis',(1.,0.,0.));
#9670=DIRECTION('center_axis',(0.,0.,-1.));
#9671=DIRECTION('ref_axis',(1.,0.,0.));
#9672=DIRECTION('center_axis',(0.,0.,-1.));
#9673=DIRECTION('ref_axis',(1.,0.,0.));
#9674=DIRECTION('center_axis',(0.,0.,1.));
#9675=DIRECTION('ref_axis',(1.,0.,0.));
#9676=DIRECTION('center_axis',(0.,0.,1.));
#9677=DIRECTION('ref_axis',(1.,0.,0.));
#9678=DIRECTION('',(0.,0.,1.));
#9679=DIRECTION('center_axis',(0.,0.,1.));
#9680=DIRECTION('ref_axis',(1.,0.,0.));
#9681=DIRECTION('center_axis',(0.,0.,1.));
#9682=DIRECTION('ref_axis',(1.,0.,0.));
#9683=DIRECTION('',(0.,0.,1.));
#9684=DIRECTION('center_axis',(0.,0.,1.));
#9685=DIRECTION('ref_axis',(1.,0.,0.));
#9686=DIRECTION('center_axis',(0.,0.,1.));
#9687=DIRECTION('ref_axis',(1.,0.,0.));
#9688=DIRECTION('',(0.,0.,1.));
#9689=DIRECTION('center_axis',(0.,0.,1.));
#9690=DIRECTION('ref_axis',(1.,0.,0.));
#9691=DIRECTION('center_axis',(0.,0.,1.));
#9692=DIRECTION('ref_axis',(1.,0.,0.));
#9693=DIRECTION('',(0.,0.,1.));
#9694=DIRECTION('center_axis',(0.,0.,1.));
#9695=DIRECTION('ref_axis',(1.,0.,0.));
#9696=DIRECTION('center_axis',(0.,0.,1.));
#9697=DIRECTION('ref_axis',(1.,0.,0.));
#9698=DIRECTION('',(0.,0.,-1.));
#9699=DIRECTION('center_axis',(0.,0.,1.));
#9700=DIRECTION('ref_axis',(1.,0.,0.));
#9701=DIRECTION('center_axis',(0.,0.,1.));
#9702=DIRECTION('ref_axis',(1.,0.,0.));
#9703=DIRECTION('',(0.,0.,1.));
#9704=DIRECTION('center_axis',(0.,0.,-1.));
#9705=DIRECTION('ref_axis',(1.,0.,0.));
#9706=DIRECTION('center_axis',(0.,0.,1.));
#9707=DIRECTION('ref_axis',(1.,0.,0.));
#9708=DIRECTION('center_axis',(0.,0.,1.));
#9709=DIRECTION('ref_axis',(1.,0.,0.));
#9710=DIRECTION('center_axis',(0.,0.,1.));
#9711=DIRECTION('ref_axis',(1.,0.,0.));
#9712=DIRECTION('',(0.,0.,-1.));
#9713=DIRECTION('center_axis',(0.,0.,1.));
#9714=DIRECTION('ref_axis',(1.,0.,0.));
#9715=DIRECTION('center_axis',(0.,0.,1.));
#9716=DIRECTION('ref_axis',(1.,0.,0.));
#9717=DIRECTION('',(0.,0.,-1.));
#9718=DIRECTION('center_axis',(0.,0.,-1.));
#9719=DIRECTION('ref_axis',(1.,0.,0.));
#9720=DIRECTION('center_axis',(0.,0.,1.));
#9721=DIRECTION('ref_axis',(1.,0.,0.));
#9722=DIRECTION('center_axis',(0.,0.,1.));
#9723=DIRECTION('ref_axis',(1.,0.,0.));
#12101=CARTESIAN_POINT('',(0.,0.,0.));
#12102=CARTESIAN_POINT('Origin',(0.9,0.,1.4));
#12103=CARTESIAN_POINT('',(0.988888264668966,0.25,1.4));
#12104=CARTESIAN_POINT('',(1.02,-1.18386380373883E-17,1.65));
#12105=CARTESIAN_POINT('Ctrl Pts',(0.988888264668966,0.25,1.4));
#12106=CARTESIAN_POINT('Ctrl Pts',(0.988888264668966,0.25,1.43153139415882));
#12107=CARTESIAN_POINT('Ctrl Pts',(0.990553370646674,0.243672048431404,
1.46507214966317));
#12108=CARTESIAN_POINT('Ctrl Pts',(0.996491737296663,0.218119830014375,
1.52662620974954));
#12109=CARTESIAN_POINT('Ctrl Pts',(1.00067109353237,0.198902128206072,1.5546512623872));
#12110=CARTESIAN_POINT('Ctrl Pts',(1.00845756932386,0.154654113568716,1.59889927702456));
#12111=CARTESIAN_POINT('Ctrl Pts',(1.01258144235289,0.126627870945253,1.61811920309393));
#12112=CARTESIAN_POINT('Ctrl Pts',(1.0183917429657,0.065069600391363,1.64367304400768));
#12113=CARTESIAN_POINT('Ctrl Pts',(1.02,0.031527330883376,1.65));
#12114=CARTESIAN_POINT('Ctrl Pts',(1.02,2.77555756156289E-17,1.65));
#12115=CARTESIAN_POINT('Ctrl Pts',(1.02,6.93889390390723E-18,1.65));
#12116=CARTESIAN_POINT('Ctrl Pts',(1.02,-0.031527330883376,1.65));
#12117=CARTESIAN_POINT('Ctrl Pts',(1.0183917429657,-0.065069600391363,1.64367304400768));
#12118=CARTESIAN_POINT('Ctrl Pts',(1.01258144235289,-0.126627870945253,
1.61811920309393));
#12119=CARTESIAN_POINT('Ctrl Pts',(1.00845756932386,-0.154654113568716,
1.59889927702456));
#12120=CARTESIAN_POINT('Ctrl Pts',(1.00067109353237,-0.198902128206072,
1.5546512623872));
#12121=CARTESIAN_POINT('Ctrl Pts',(0.996491737296663,-0.218119830014375,
1.52662620974954));
#12122=CARTESIAN_POINT('Ctrl Pts',(0.990553370646674,-0.243672048431404,
1.46507214966317));
#12123=CARTESIAN_POINT('Ctrl Pts',(0.988888264668967,-0.25,1.43153139415882));
#12124=CARTESIAN_POINT('Ctrl Pts',(0.988888264668967,-0.25,1.36846860584118));
#12125=CARTESIAN_POINT('Ctrl Pts',(0.990553370646674,-0.243672048431404,
1.33492785033683));
#12126=CARTESIAN_POINT('Ctrl Pts',(0.996491737296663,-0.218119830014375,
1.27337379025046));
#12127=CARTESIAN_POINT('Ctrl Pts',(1.00067109353237,-0.198902128206072,
1.2453487376128));
#12128=CARTESIAN_POINT('Ctrl Pts',(1.00845756932386,-0.154654113568716,
1.20110072297544));
#12129=CARTESIAN_POINT('Ctrl Pts',(1.01258144235289,-0.126627870945254,
1.18188079690607));
#12130=CARTESIAN_POINT('Ctrl Pts',(1.0183917429657,-0.0650696003913633,
1.15632695599232));
#12131=CARTESIAN_POINT('Ctrl Pts',(1.02,-0.0315273308833761,1.15));
#12132=CARTESIAN_POINT('Ctrl Pts',(1.02,0.0315273308833759,1.15));
#12133=CARTESIAN_POINT('Ctrl Pts',(1.0183917429657,0.065069600391363,1.15632695599232));
#12134=CARTESIAN_POINT('Ctrl Pts',(1.01258144235289,0.126627870945253,1.18188079690607));
#12135=CARTESIAN_POINT('Ctrl Pts',(1.00845756932386,0.154654113568716,1.20110072297544));
#12136=CARTESIAN_POINT('Ctrl Pts',(1.00067109353237,0.198902128206072,1.2453487376128));
#12137=CARTESIAN_POINT('Ctrl Pts',(0.996491737296663,0.218119830014375,
1.27337379025046));
#12138=CARTESIAN_POINT('Ctrl Pts',(0.990553370646674,0.243672048431404,
1.33492785033683));
#12139=CARTESIAN_POINT('Ctrl Pts',(0.988888264668967,0.25,1.36846860584118));
#12140=CARTESIAN_POINT('Ctrl Pts',(0.988888264668967,0.25,1.4));
#12141=CARTESIAN_POINT('',(2.9,-3.06161699786838E-17,1.65));
#12142=CARTESIAN_POINT('',(0.9,-3.06161699786838E-17,1.65));
#12143=CARTESIAN_POINT('',(2.88920404263873,0.25,1.4));
#12144=CARTESIAN_POINT('Ctrl Pts',(2.88920404263873,0.25,1.4));
#12145=CARTESIAN_POINT('Ctrl Pts',(2.88920404263873,0.25,1.36859268214333));
#12146=CARTESIAN_POINT('Ctrl Pts',(2.8897689135262,0.243720046736958,1.33510260402868));
#12147=CARTESIAN_POINT('Ctrl Pts',(2.89180770664292,0.218201792012593,1.27351240469396));
#12148=CARTESIAN_POINT('Ctrl Pts',(2.89325203146722,0.198964344197684,1.24541095360441));
#12149=CARTESIAN_POINT('Ctrl Pts',(2.89596207500507,0.154589088004924,1.20103569741165));
#12150=CARTESIAN_POINT('Ctrl Pts',(2.89740405468483,0.126487618562645,1.18179821727709));
#12151=CARTESIAN_POINT('Ctrl Pts',(2.89943748106926,0.0648973582672708,
1.15627993798745));
#12152=CARTESIAN_POINT('Ctrl Pts',(2.9,0.0314072589573412,1.15));
#12153=CARTESIAN_POINT('Ctrl Pts',(2.9,-0.0314072589573412,1.15));
#12154=CARTESIAN_POINT('Ctrl Pts',(2.89943748106926,-0.0648973582672708,
1.15627993798745));
#12155=CARTESIAN_POINT('Ctrl Pts',(2.89740405468483,-0.126487618562645,
1.18179821727709));
#12156=CARTESIAN_POINT('Ctrl Pts',(2.89596207500507,-0.154589088004924,
1.20103569741165));
#12157=CARTESIAN_POINT('Ctrl Pts',(2.89325203146722,-0.198964344197684,
1.24541095360441));
#12158=CARTESIAN_POINT('Ctrl Pts',(2.89180770664292,-0.218201792012593,
1.27351240469396));
#12159=CARTESIAN_POINT('Ctrl Pts',(2.8897689135262,-0.243720046736958,1.33510260402868));
#12160=CARTESIAN_POINT('Ctrl Pts',(2.88920404263873,-0.25,1.36859268214333));
#12161=CARTESIAN_POINT('Ctrl Pts',(2.88920404263873,-0.25,1.43140731785667));
#12162=CARTESIAN_POINT('Ctrl Pts',(2.8897689135262,-0.243720046736958,1.46489739597132));
#12163=CARTESIAN_POINT('Ctrl Pts',(2.89180770664292,-0.218201792012593,
1.52648759530604));
#12164=CARTESIAN_POINT('Ctrl Pts',(2.89325203146722,-0.198964344197684,
1.55458904639559));
#12165=CARTESIAN_POINT('Ctrl Pts',(2.89596207500507,-0.154589088004924,
1.59896430258835));
#12166=CARTESIAN_POINT('Ctrl Pts',(2.89740405468483,-0.126487618562645,
1.61820178272291));
#12167=CARTESIAN_POINT('Ctrl Pts',(2.89943748106926,-0.0648973582672709,
1.64372006201255));
#12168=CARTESIAN_POINT('Ctrl Pts',(2.9,-0.0314072589573412,1.65));
#12169=CARTESIAN_POINT('Ctrl Pts',(2.9,1.38777878078145E-17,1.65));
#12170=CARTESIAN_POINT('Ctrl Pts',(2.9,-2.08166817117217E-17,1.65));
#12171=CARTESIAN_POINT('Ctrl Pts',(2.9,0.0314072589573412,1.65));
#12172=CARTESIAN_POINT('Ctrl Pts',(2.89943748106926,0.0648973582672708,
1.64372006201255));
#12173=CARTESIAN_POINT('Ctrl Pts',(2.89740405468483,0.126487618562645,1.61820178272291));
#12174=CARTESIAN_POINT('Ctrl Pts',(2.89596207500507,0.154589088004924,1.59896430258835));
#12175=CARTESIAN_POINT('Ctrl Pts',(2.89325203146722,0.198964344197684,1.55458904639559));
#12176=CARTESIAN_POINT('Ctrl Pts',(2.89180770664292,0.218201792012593,1.52648759530604));
#12177=CARTESIAN_POINT('Ctrl Pts',(2.8897689135262,0.243720046736958,1.46489739597132));
#12178=CARTESIAN_POINT('Ctrl Pts',(2.88920404263873,0.25,1.43140731785667));
#12179=CARTESIAN_POINT('Ctrl Pts',(2.88920404263873,0.25,1.4));
#12180=CARTESIAN_POINT('Origin',(-1.23743686707646,-1.23743686707646,2.9));
#12181=CARTESIAN_POINT('',(-1.40243686707646,-1.23743686707646,2.9));
#12182=CARTESIAN_POINT('Origin',(-1.23743686707646,-1.23743686707646,2.9));
#12183=CARTESIAN_POINT('',(-1.40243686707646,-1.23743686707646,3.6));
#12184=CARTESIAN_POINT('',(-1.40243686707646,-1.23743686707646,2.9));
#12185=CARTESIAN_POINT('Origin',(-1.23743686707646,-1.23743686707646,3.6));
#12186=CARTESIAN_POINT('Origin',(-1.23743686707646,-1.23743686707646,2.9));
#12187=CARTESIAN_POINT('Origin',(-1.23743686707646,1.23743686707646,2.9));
#12188=CARTESIAN_POINT('',(-1.40243686707646,1.23743686707646,2.9));
#12189=CARTESIAN_POINT('Origin',(-1.23743686707646,1.23743686707646,2.9));
#12190=CARTESIAN_POINT('',(-1.40243686707646,1.23743686707646,3.6));
#12191=CARTESIAN_POINT('',(-1.40243686707646,1.23743686707646,2.9));
#12192=CARTESIAN_POINT('Origin',(-1.23743686707646,1.23743686707646,3.6));
#12193=CARTESIAN_POINT('Origin',(-1.23743686707646,1.23743686707646,2.9));
#12194=CARTESIAN_POINT('Origin',(1.23743686707646,1.23743686707646,2.9));
#12195=CARTESIAN_POINT('',(1.07243686707646,1.23743686707646,2.9));
#12196=CARTESIAN_POINT('Origin',(1.23743686707646,1.23743686707646,2.9));
#12197=CARTESIAN_POINT('',(1.07243686707646,1.23743686707646,3.6));
#12198=CARTESIAN_POINT('',(1.07243686707646,1.23743686707646,2.9));
#12199=CARTESIAN_POINT('Origin',(1.23743686707646,1.23743686707646,3.6));
#12200=CARTESIAN_POINT('Origin',(1.23743686707646,1.23743686707646,2.9));
#12201=CARTESIAN_POINT('Origin',(1.23743686707646,-1.23743686707646,2.9));
#12202=CARTESIAN_POINT('',(1.07243686707646,-1.23743686707646,2.9));
#12203=CARTESIAN_POINT('Origin',(1.23743686707646,-1.23743686707646,2.9));
#12204=CARTESIAN_POINT('',(1.07243686707646,-1.23743686707646,3.6));
#12205=CARTESIAN_POINT('',(1.07243686707646,-1.23743686707646,2.9));
#12206=CARTESIAN_POINT('Origin',(1.23743686707646,-1.23743686707646,3.6));
#12207=CARTESIAN_POINT('Origin',(1.23743686707646,-1.23743686707646,2.9));
#12208=CARTESIAN_POINT('Origin',(-1.69705627484771,-1.69705627484771,1.8));
#12209=CARTESIAN_POINT('',(-1.19413676298012,-1.84771139285857,2.4));
#12210=CARTESIAN_POINT('',(-1.19413676298012,-1.84771139285857,1.8));
#12211=CARTESIAN_POINT('',(-1.19413676298012,-1.84771139285857,1.8));
#12212=CARTESIAN_POINT('',(-1.84771139285857,-1.19413676298012,2.4));
#12213=CARTESIAN_POINT('Origin',(-1.69705627484771,-1.69705627484771,2.4));
#12214=CARTESIAN_POINT('',(-1.84771139285857,-1.19413676298012,1.8));
#12215=CARTESIAN_POINT('',(-1.84771139285857,-1.19413676298012,1.8));
#12216=CARTESIAN_POINT('Origin',(-1.69705627484771,-1.69705627484771,1.8));
#12217=CARTESIAN_POINT('Origin',(-1.69705627484771,-1.69705627484771,2.4));
#12218=CARTESIAN_POINT('Origin',(0.,0.,2.4));
#12219=CARTESIAN_POINT('Origin',(-1.69705627484771,1.69705627484771,1.8));
#12220=CARTESIAN_POINT('',(-1.84771139285857,1.19413676298012,2.4));
#12221=CARTESIAN_POINT('',(-1.84771139285857,1.19413676298012,1.8));
#12222=CARTESIAN_POINT('',(-1.84771139285857,1.19413676298012,1.8));
#12223=CARTESIAN_POINT('',(-1.19413676298012,1.84771139285857,2.4));
#12224=CARTESIAN_POINT('Origin',(-1.69705627484771,1.69705627484771,2.4));
#12225=CARTESIAN_POINT('',(-1.19413676298012,1.84771139285857,1.8));
#12226=CARTESIAN_POINT('',(-1.19413676298012,1.84771139285857,1.8));
#12227=CARTESIAN_POINT('Origin',(-1.69705627484771,1.69705627484771,1.8));
#12228=CARTESIAN_POINT('Origin',(-1.69705627484771,1.69705627484771,2.4));
#12229=CARTESIAN_POINT('Origin',(0.,0.,2.4));
#12230=CARTESIAN_POINT('Origin',(1.69705627484771,1.69705627484771,1.8));
#12231=CARTESIAN_POINT('',(1.19413676298012,1.84771139285857,2.4));
#12232=CARTESIAN_POINT('',(1.19413676298012,1.84771139285857,1.8));
#12233=CARTESIAN_POINT('',(1.19413676298012,1.84771139285857,1.8));
#12234=CARTESIAN_POINT('',(1.84771139285857,1.19413676298012,2.4));
#12235=CARTESIAN_POINT('Origin',(1.69705627484771,1.69705627484771,2.4));
#12236=CARTESIAN_POINT('',(1.84771139285857,1.19413676298012,1.8));
#12237=CARTESIAN_POINT('',(1.84771139285857,1.19413676298012,1.8));
#12238=CARTESIAN_POINT('Origin',(1.69705627484771,1.69705627484771,1.8));
#12239=CARTESIAN_POINT('Origin',(1.69705627484771,1.69705627484771,2.4));
#12240=CARTESIAN_POINT('Origin',(0.,0.,2.4));
#12241=CARTESIAN_POINT('Origin',(1.69705627484771,-1.69705627484771,1.8));
#12242=CARTESIAN_POINT('',(1.84771139285857,-1.19413676298012,2.4));
#12243=CARTESIAN_POINT('',(1.84771139285857,-1.19413676298012,1.8));
#12244=CARTESIAN_POINT('',(1.84771139285857,-1.19413676298012,1.8));
#12245=CARTESIAN_POINT('',(1.19413676298012,-1.84771139285857,2.4));
#12246=CARTESIAN_POINT('Origin',(1.69705627484771,-1.69705627484771,2.4));
#12247=CARTESIAN_POINT('',(1.19413676298012,-1.84771139285857,1.8));
#12248=CARTESIAN_POINT('',(1.19413676298012,-1.84771139285857,1.8));
#12249=CARTESIAN_POINT('Origin',(1.69705627484771,-1.69705627484771,1.8));
#12250=CARTESIAN_POINT('Origin',(1.69705627484771,-1.69705627484771,2.4));
#12251=CARTESIAN_POINT('Origin',(0.,0.,2.4));
#12252=CARTESIAN_POINT('Origin',(0.,0.,1.8));
#12253=CARTESIAN_POINT('',(-2.9,-3.55147571752732E-16,1.8));
#12254=CARTESIAN_POINT('Origin',(0.,0.,1.8));
#12255=CARTESIAN_POINT('',(-2.2,-2.69422295812418E-16,1.8));
#12256=CARTESIAN_POINT('Origin',(0.,0.,1.8));
#12257=CARTESIAN_POINT('Origin',(0.,0.,1.8));
#12258=CARTESIAN_POINT('Origin',(0.,0.,1.8));
#12259=CARTESIAN_POINT('Origin',(0.,0.,1.8));
#12260=CARTESIAN_POINT('Origin',(0.,0.,1.8));
#12261=CARTESIAN_POINT('',(-1.97205627484771,-1.69705627484771,1.8));
#12262=CARTESIAN_POINT('Origin',(-1.69705627484771,-1.69705627484771,1.8));
#12263=CARTESIAN_POINT('',(-1.97205627484771,1.69705627484771,1.8));
#12264=CARTESIAN_POINT('Origin',(-1.69705627484771,1.69705627484771,1.8));
#12265=CARTESIAN_POINT('',(1.42205627484771,1.69705627484771,1.8));
#12266=CARTESIAN_POINT('Origin',(1.69705627484771,1.69705627484771,1.8));
#12267=CARTESIAN_POINT('',(1.42205627484771,-1.69705627484771,1.8));
#12268=CARTESIAN_POINT('Origin',(1.69705627484771,-1.69705627484771,1.8));
#12269=CARTESIAN_POINT('Origin',(-1.69705627484771,-1.69705627484771,0.9));
#12270=CARTESIAN_POINT('',(-1.97205627484771,-1.69705627484771,1.));
#12271=CARTESIAN_POINT('Origin',(-1.69705627484771,-1.69705627484771,1.));
#12272=CARTESIAN_POINT('',(-1.97205627484771,-1.69705627484771,0.9));
#12273=CARTESIAN_POINT('Origin',(-1.69705627484771,1.69705627484771,0.9));
#12274=CARTESIAN_POINT('',(-1.97205627484771,1.69705627484771,1.));
#12275=CARTESIAN_POINT('Origin',(-1.69705627484771,1.69705627484771,1.));
#12276=CARTESIAN_POINT('',(-1.97205627484771,1.69705627484771,0.9));
#12277=CARTESIAN_POINT('Origin',(1.69705627484771,1.69705627484771,0.9));
#12278=CARTESIAN_POINT('',(1.42205627484771,1.69705627484771,1.));
#12279=CARTESIAN_POINT('Origin',(1.69705627484771,1.69705627484771,1.));
#12280=CARTESIAN_POINT('',(1.42205627484771,1.69705627484771,0.9));
#12281=CARTESIAN_POINT('Origin',(1.69705627484771,-1.69705627484771,0.9));
#12282=CARTESIAN_POINT('',(1.42205627484771,-1.69705627484771,1.));
#12283=CARTESIAN_POINT('Origin',(1.69705627484771,-1.69705627484771,1.));
#12284=CARTESIAN_POINT('',(1.42205627484771,-1.69705627484771,0.9));
#12285=CARTESIAN_POINT('Origin',(0.,0.,1.));
#12286=CARTESIAN_POINT('',(-2.2,-2.69422295812418E-16,3.6));
#12287=CARTESIAN_POINT('Origin',(0.,0.,3.6));
#12288=CARTESIAN_POINT('',(-2.2,-2.69422295812418E-16,1.));
#12289=CARTESIAN_POINT('Origin',(0.,0.,2.05));
#12290=CARTESIAN_POINT('',(-1.5,-1.83697019872103E-16,2.05));
#12291=CARTESIAN_POINT('Origin',(0.,0.,2.05));
#12292=CARTESIAN_POINT('',(-1.5,1.83697019872103E-16,3.6));
#12293=CARTESIAN_POINT('',(-1.5,-1.83697019872103E-16,2.05));
#12294=CARTESIAN_POINT('Origin',(0.,0.,3.6));
#12295=CARTESIAN_POINT('Origin',(0.,0.,2.05));
#12296=CARTESIAN_POINT('',(-1.02,-1.2491397351303E-16,2.05));
#12297=CARTESIAN_POINT('Origin',(0.,0.,2.05));
#12298=CARTESIAN_POINT('Origin',(0.,0.,1.));
#12299=CARTESIAN_POINT('',(-2.9,-3.55147571752732E-16,1.));
#12300=CARTESIAN_POINT('',(-2.9,-3.55147571752732E-16,1.));
#12301=CARTESIAN_POINT('Origin',(0.,0.,1.));
#12302=CARTESIAN_POINT('Origin',(0.,0.,1.));
#12303=CARTESIAN_POINT('',(-1.02,-1.2491397351303E-16,1.));
#12304=CARTESIAN_POINT('',(-1.02,-1.2491397351303E-16,1.));
#12305=CARTESIAN_POINT('Origin',(0.,0.,1.));
#12306=CARTESIAN_POINT('Origin',(0.,0.,3.6));
#12307=CARTESIAN_POINT('Origin',(0.,0.,1.));
#14776=UNCERTAINTY_MEASURE_WITH_UNIT(LENGTH_MEASURE(0.001),#14879,
'DISTANCE_ACCURACY_VALUE',
'Maximum model space distance between geometric entities at asserted c
onnectivities');
#14824=UNCERTAINTY_MEASURE_WITH_UNIT(LENGTH_MEASURE(0.001),#14879,
'DISTANCE_ACCURACY_VALUE',
'Maximum model space distance between geometric entities at asserted c
onnectivities');
#14830=(
GEOMETRIC_REPRESENTATION_CONTEXT(3)
GLOBAL_UNCERTAINTY_ASSIGNED_CONTEXT((#14776))
GLOBAL_UNIT_ASSIGNED_CONTEXT((#14879,#14881,#14882))
REPRESENTATION_CONTEXT('','3D')
);
#14878=(
GEOMETRIC_REPRESENTATION_CONTEXT(3)
GLOBAL_UNCERTAINTY_ASSIGNED_CONTEXT((#14824))
GLOBAL_UNIT_ASSIGNED_CONTEXT((#14879,#14881,#14882))
REPRESENTATION_CONTEXT('','3D')
);
#14879=(
LENGTH_UNIT()
NAMED_UNIT(*)
SI_UNIT(.CENTI.,.METRE.)
);
#14881=(
NAMED_UNIT(*)
PLANE_ANGLE_UNIT()
SI_UNIT($,.RADIAN.)
);
#14882=(
NAMED_UNIT(*)
SI_UNIT($,.STERADIAN.)
SOLID_ANGLE_UNIT()
);
#14888=SHAPE_DEFINITION_REPRESENTATION(#14941,#15073);
#14941=PRODUCT_DEFINITION_SHAPE('',$,#15127);
#15073=SHAPE_REPRESENTATION('',(#8443),#14830);
#15121=PRODUCT_DEFINITION_CONTEXT('part definition',#15282,'design');
#15127=PRODUCT_DEFINITION('Lever bearing post','Lever bearing post',#15180,
#15121);
#15180=PRODUCT_DEFINITION_FORMATION('',$,#15289);
#15282=APPLICATION_CONTEXT(
'Core Data for Automotive Mechanical Design Process');
#15283=PRODUCT_CONTEXT('part definition',#15282,'mechanical');
#15289=PRODUCT('Lever bearing post','Lever bearing post',
'Lever bearing post',(#15283));
#15400=COLOUR_RGB('Grey',0.48,0.52,0.57);
#15401=FILL_AREA_STYLE_COLOUR('',#15400);
#15402=FILL_AREA_STYLE('',(#15401));
#15403=SURFACE_STYLE_FILL_AREA(#15402);
#15404=SURFACE_SIDE_STYLE('',(#15403));
#15405=SURFACE_STYLE_USAGE(.BOTH.,#15404);
#15406=PRESENTATION_STYLE_ASSIGNMENT((#15405));
ENDSEC;
END-ISO-10303-21;
